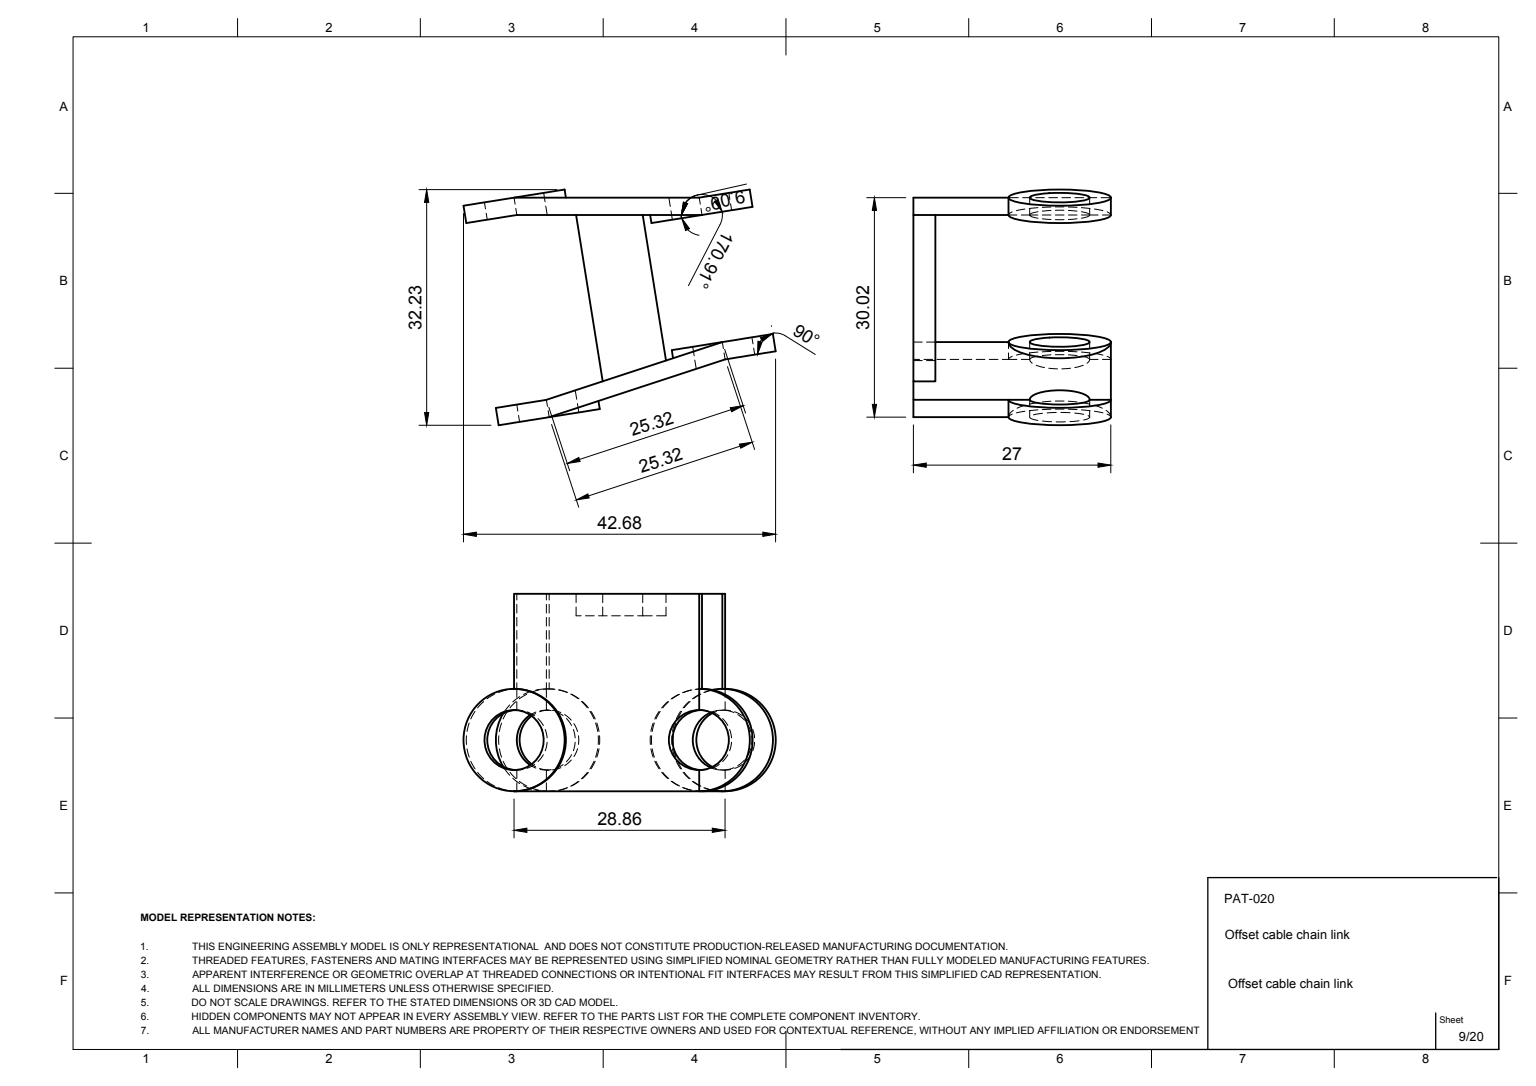
ISO-10303-21;
HEADER;
/* Generated by software containing ST-Developer
 * from STEP Tools, Inc. (www.steptools.com) 
 */

FILE_DESCRIPTION(
/* description */ ('Cable chain and bracket set'),
/* implementation_level */ '2;1');

FILE_NAME(
/* name */ 'Offset cable chain link.step',
/* time_stamp */ '2026-10-29T17:19:47-07:00',
/* author */ (''),
/* organization */ (''),
/* preprocessor_version */ 'ST-DEVELOPER v20.2',
/* originating_system */ 'Autodesk Translation Framework v15.17.0.0',
/* authorisation */ '');

FILE_SCHEMA (('AUTOMOTIVE_DESIGN { 1 0 10303 214 3 1 1 }'));
ENDSEC;

DATA;
#10=MECHANICAL_DESIGN_GEOMETRIC_PRESENTATION_REPRESENTATION('',(#338),#5929);
#291=ELLIPSE('',#3464,0.415214835958494,0.410000000000047);
#292=ELLIPSE('',#3467,0.415214835958494,0.410000000000047);
#293=ELLIPSE('',#3473,0.415214835958495,0.410000000000047);
#294=ELLIPSE('',#3475,0.415214835958495,0.410000000000047);
#295=ELLIPSE('',#3478,0.415214835958495,0.410000000000047);
#296=ELLIPSE('',#3480,0.415214835958495,0.410000000000047);
#297=ELLIPSE('',#3486,0.708903378465722,0.70000000000008);
#298=ELLIPSE('',#3488,0.708903378465722,0.70000000000008);
#299=ELLIPSE('',#3499,0.708903378465722,0.70000000000008);
#300=ELLIPSE('',#3510,0.708903378465722,0.70000000000008);
#312=SHAPE_REPRESENTATION_RELATIONSHIP('SRR','None',#6043,#325);
#325=ADVANCED_BREP_SHAPE_REPRESENTATION('',(#351),#5910);
#338=STYLED_ITEM('',(#6234),#351);
#351=MANIFOLD_SOLID_BREP('Body1',#3332);
#371=FACE_BOUND('',#751,.T.);
#372=FACE_BOUND('',#762,.T.);
#373=FACE_BOUND('',#765,.T.);
#374=FACE_BOUND('',#774,.T.);
#421=PLANE('',#3481);
#422=PLANE('',#3483);
#423=PLANE('',#3485);
#424=PLANE('',#3487);
#425=PLANE('',#3489);
#426=PLANE('',#3490);
#427=PLANE('',#3491);
#428=PLANE('',#3492);
#429=PLANE('',#3497);
#430=PLANE('',#3500);
#431=PLANE('',#3501);
#432=PLANE('',#3502);
#433=PLANE('',#3503);
#434=PLANE('',#3508);
#435=PLANE('',#3509);
#436=PLANE('',#3511);
#437=PLANE('',#3517);
#438=PLANE('',#3518);
#439=PLANE('',#3519);
#440=PLANE('',#3520);
#441=PLANE('',#3521);
#442=PLANE('',#3522);
#549=FACE_OUTER_BOUND('',#739,.T.);
#550=FACE_OUTER_BOUND('',#740,.T.);
#551=FACE_OUTER_BOUND('',#741,.T.);
#552=FACE_OUTER_BOUND('',#742,.T.);
#553=FACE_OUTER_BOUND('',#743,.T.);
#554=FACE_OUTER_BOUND('',#744,.T.);
#555=FACE_OUTER_BOUND('',#745,.T.);
#556=FACE_OUTER_BOUND('',#746,.T.);
#557=FACE_OUTER_BOUND('',#747,.T.);
#558=FACE_OUTER_BOUND('',#748,.T.);
#559=FACE_OUTER_BOUND('',#749,.T.);
#560=FACE_OUTER_BOUND('',#750,.T.);
#561=FACE_OUTER_BOUND('',#752,.T.);
#562=FACE_OUTER_BOUND('',#753,.T.);
#563=FACE_OUTER_BOUND('',#754,.T.);
#564=FACE_OUTER_BOUND('',#755,.T.);
#565=FACE_OUTER_BOUND('',#756,.T.);
#566=FACE_OUTER_BOUND('',#757,.T.);
#567=FACE_OUTER_BOUND('',#758,.T.);
#568=FACE_OUTER_BOUND('',#759,.T.);
#569=FACE_OUTER_BOUND('',#760,.T.);
#570=FACE_OUTER_BOUND('',#761,.T.);
#571=FACE_OUTER_BOUND('',#763,.T.);
#572=FACE_OUTER_BOUND('',#764,.T.);
#573=FACE_OUTER_BOUND('',#766,.T.);
#574=FACE_OUTER_BOUND('',#767,.T.);
#575=FACE_OUTER_BOUND('',#768,.T.);
#576=FACE_OUTER_BOUND('',#769,.T.);
#577=FACE_OUTER_BOUND('',#770,.T.);
#578=FACE_OUTER_BOUND('',#771,.T.);
#579=FACE_OUTER_BOUND('',#772,.T.);
#580=FACE_OUTER_BOUND('',#773,.T.);
#581=FACE_OUTER_BOUND('',#775,.T.);
#582=FACE_OUTER_BOUND('',#776,.T.);
#739=EDGE_LOOP('',(#2369,#2370,#2371,#2372,#2373,#2374));
#740=EDGE_LOOP('',(#2375,#2376,#2377,#2378,#2379,#2380));
#741=EDGE_LOOP('',(#2381,#2382,#2383,#2384,#2385,#2386));
#742=EDGE_LOOP('',(#2387,#2388,#2389,#2390,#2391,#2392));
#743=EDGE_LOOP('',(#2393,#2394,#2395,#2396,#2397));
#744=EDGE_LOOP('',(#2398,#2399,#2400,#2401,#2402));
#745=EDGE_LOOP('',(#2403,#2404,#2405,#2406,#2407,#2408,#2409,#2410,#2411));
#746=EDGE_LOOP('',(#2412,#2413,#2414,#2415,#2416,#2417,#2418,#2419,#2420));
#747=EDGE_LOOP('',(#2421,#2422,#2423,#2424));
#748=EDGE_LOOP('',(#2425,#2426,#2427,#2428));
#749=EDGE_LOOP('',(#2429,#2430,#2431,#2432));
#750=EDGE_LOOP('',(#2433,#2434));
#751=EDGE_LOOP('',(#2435));
#752=EDGE_LOOP('',(#2436,#2437,#2438,#2439));
#753=EDGE_LOOP('',(#2440,#2441,#2442,#2443));
#754=EDGE_LOOP('',(#2444,#2445));
#755=EDGE_LOOP('',(#2446,#2447,#2448,#2449,#2450,#2451,#2452,#2453,#2454,
#2455,#2456,#2457));
#756=EDGE_LOOP('',(#2458,#2459,#2460,#2461));
#757=EDGE_LOOP('',(#2462,#2463,#2464,#2465));
#758=EDGE_LOOP('',(#2466,#2467,#2468,#2469));
#759=EDGE_LOOP('',(#2470,#2471));
#760=EDGE_LOOP('',(#2472,#2473,#2474,#2475));
#761=EDGE_LOOP('',(#2476,#2477));
#762=EDGE_LOOP('',(#2478));
#763=EDGE_LOOP('',(#2479,#2480,#2481,#2482,#2483,#2484,#2485,#2486,#2487,
#2488,#2489,#2490));
#764=EDGE_LOOP('',(#2491,#2492));
#765=EDGE_LOOP('',(#2493));
#766=EDGE_LOOP('',(#2494,#2495));
#767=EDGE_LOOP('',(#2496,#2497,#2498,#2499));
#768=EDGE_LOOP('',(#2500,#2501,#2502,#2503));
#769=EDGE_LOOP('',(#2504,#2505,#2506,#2507));
#770=EDGE_LOOP('',(#2508,#2509,#2510,#2511));
#771=EDGE_LOOP('',(#2512,#2513,#2514,#2515));
#772=EDGE_LOOP('',(#2516,#2517,#2518,#2519,#2520,#2521,#2522,#2523,#2524,
#2525,#2526,#2527));
#773=EDGE_LOOP('',(#2528,#2529));
#774=EDGE_LOOP('',(#2530));
#775=EDGE_LOOP('',(#2531,#2532));
#776=EDGE_LOOP('',(#2533,#2534,#2535,#2536));
#981=LINE('',#4989,#1241);
#982=LINE('',#5002,#1242);
#983=LINE('',#5012,#1243);
#984=LINE('',#5019,#1244);
#985=LINE('',#5027,#1245);
#986=LINE('',#5030,#1246);
#987=LINE('',#5033,#1247);
#988=LINE('',#5036,#1248);
#989=LINE('',#5039,#1249);
#990=LINE('',#5041,#1250);
#991=LINE('',#5043,#1251);
#992=LINE('',#5045,#1252);
#993=LINE('',#5049,#1253);
#994=LINE('',#5050,#1254);
#995=LINE('',#5053,#1255);
#996=LINE('',#5055,#1256);
#997=LINE('',#5059,#1257);
#998=LINE('',#5061,#1258);
#999=LINE('',#5063,#1259);
#1000=LINE('',#5064,#1260);
#1001=LINE('',#5068,#1261);
#1002=LINE('',#5070,#1262);
#1003=LINE('',#5072,#1263);
#1004=LINE('',#5073,#1264);
#1005=LINE('',#5077,#1265);
#1006=LINE('',#5079,#1266);
#1007=LINE('',#5081,#1267);
#1008=LINE('',#5082,#1268);
#1009=LINE('',#5084,#1269);
#1010=LINE('',#5085,#1270);
#1011=LINE('',#5092,#1271);
#1012=LINE('',#5094,#1272);
#1013=LINE('',#5100,#1273);
#1014=LINE('',#5101,#1274);
#1015=LINE('',#5103,#1275);
#1016=LINE('',#5104,#1276);
#1017=LINE('',#5105,#1277);
#1018=LINE('',#5107,#1278);
#1019=LINE('',#5109,#1279);
#1020=LINE('',#5110,#1280);
#1021=LINE('',#5112,#1281);
#1022=LINE('',#5120,#1282);
#1023=LINE('',#5124,#1283);
#1024=LINE('',#5125,#1284);
#1025=LINE('',#5127,#1285);
#1026=LINE('',#5128,#1286);
#1027=LINE('',#5134,#1287);
#1028=LINE('',#5135,#1288);
#1029=LINE('',#5139,#1289);
#1030=LINE('',#5141,#1290);
#1031=LINE('',#5142,#1291);
#1032=LINE('',#5144,#1292);
#1241=VECTOR('',#3944,0.410000000000047);
#1242=VECTOR('',#3957,0.410000000000047);
#1243=VECTOR('',#3968,0.410000000000047);
#1244=VECTOR('',#3977,0.410000000000047);
#1245=VECTOR('',#3986,1.00000000000011);
#1246=VECTOR('',#3989,1.00000000000011);
#1247=VECTOR('',#3992,1.00000000000011);
#1248=VECTOR('',#3995,1.00000000000011);
#1249=VECTOR('',#3998,1.00000000000011);
#1250=VECTOR('',#3999,1.00000000000011);
#1251=VECTOR('',#4000,1.00000000000011);
#1252=VECTOR('',#4001,1.00000000000011);
#1253=VECTOR('',#4004,1.00000000000011);
#1254=VECTOR('',#4005,1.00000000000011);
#1255=VECTOR('',#4008,1.00000000000011);
#1256=VECTOR('',#4009,1.00000000000011);
#1257=VECTOR('',#4012,1.00000000000011);
#1258=VECTOR('',#4013,1.00000000000011);
#1259=VECTOR('',#4014,1.00000000000011);
#1260=VECTOR('',#4015,1.00000000000011);
#1261=VECTOR('',#4018,1.00000000000011);
#1262=VECTOR('',#4019,1.00000000000011);
#1263=VECTOR('',#4020,1.00000000000011);
#1264=VECTOR('',#4021,1.00000000000011);
#1265=VECTOR('',#4024,1.00000000000011);
#1266=VECTOR('',#4025,1.00000000000011);
#1267=VECTOR('',#4026,1.00000000000011);
#1268=VECTOR('',#4027,1.00000000000011);
#1269=VECTOR('',#4030,1.00000000000011);
#1270=VECTOR('',#4031,1.00000000000011);
#1271=VECTOR('',#4040,1.00000000000011);
#1272=VECTOR('',#4043,1.00000000000011);
#1273=VECTOR('',#4052,1.00000000000011);
#1274=VECTOR('',#4053,1.00000000000011);
#1275=VECTOR('',#4054,1.00000000000011);
#1276=VECTOR('',#4055,1.00000000000011);
#1277=VECTOR('',#4056,1.00000000000011);
#1278=VECTOR('',#4059,1.00000000000011);
#1279=VECTOR('',#4062,1.00000000000011);
#1280=VECTOR('',#4063,1.00000000000011);
#1281=VECTOR('',#4066,1.00000000000011);
#1282=VECTOR('',#4079,1.00000000000011);
#1283=VECTOR('',#4082,1.00000000000011);
#1284=VECTOR('',#4083,1.00000000000011);
#1285=VECTOR('',#4084,1.00000000000011);
#1286=VECTOR('',#4085,1.00000000000011);
#1287=VECTOR('',#4096,1.00000000000011);
#1288=VECTOR('',#4097,1.00000000000011);
#1289=VECTOR('',#4104,1.00000000000011);
#1290=VECTOR('',#4107,1.00000000000011);
#1291=VECTOR('',#4108,1.00000000000011);
#1292=VECTOR('',#4111,1.00000000000011);
#1465=CIRCLE('',#3462,0.410000000000047);
#1466=CIRCLE('',#3463,0.410000000000047);
#1467=CIRCLE('',#3465,0.410000000000047);
#1468=CIRCLE('',#3468,0.410000000000047);
#1469=CIRCLE('',#3469,0.410000000000047);
#1470=CIRCLE('',#3470,0.410000000000047);
#1471=CIRCLE('',#3472,0.410000000000047);
#1472=CIRCLE('',#3474,0.410000000000047);
#1473=CIRCLE('',#3477,0.410000000000047);
#1474=CIRCLE('',#3479,0.410000000000047);
#1475=CIRCLE('',#3482,0.70000000000008);
#1476=CIRCLE('',#3484,0.70000000000008);
#1477=CIRCLE('',#3493,0.70000000000008);
#1478=CIRCLE('',#3494,0.70000000000008);
#1479=CIRCLE('',#3496,0.70000000000008);
#1480=CIRCLE('',#3505,0.70000000000008);
#1481=CIRCLE('',#3507,0.70000000000008);
#1482=CIRCLE('',#3512,0.70000000000008);
#1483=CIRCLE('',#3513,0.70000000000008);
#1484=CIRCLE('',#3516,0.70000000000008);
#1485=CIRCLE('',#3523,0.70000000000008);
#1486=CIRCLE('',#3524,0.70000000000008);
#1601=VERTEX_POINT('',#4986);
#1602=VERTEX_POINT('',#4988);
#1603=VERTEX_POINT('',#4990);
#1604=VERTEX_POINT('',#4992);
#1605=VERTEX_POINT('',#4996);
#1606=VERTEX_POINT('',#4997);
#1607=VERTEX_POINT('',#4999);
#1608=VERTEX_POINT('',#5001);
#1609=VERTEX_POINT('',#5006);
#1610=VERTEX_POINT('',#5007);
#1611=VERTEX_POINT('',#5009);
#1612=VERTEX_POINT('',#5011);
#1613=VERTEX_POINT('',#5016);
#1614=VERTEX_POINT('',#5018);
#1615=VERTEX_POINT('',#5020);
#1616=VERTEX_POINT('',#5022);
#1617=VERTEX_POINT('',#5026);
#1618=VERTEX_POINT('',#5028);
#1619=VERTEX_POINT('',#5032);
#1620=VERTEX_POINT('',#5034);
#1621=VERTEX_POINT('',#5038);
#1622=VERTEX_POINT('',#5040);
#1623=VERTEX_POINT('',#5042);
#1624=VERTEX_POINT('',#5044);
#1625=VERTEX_POINT('',#5046);
#1626=VERTEX_POINT('',#5048);
#1627=VERTEX_POINT('',#5052);
#1628=VERTEX_POINT('',#5054);
#1629=VERTEX_POINT('',#5056);
#1630=VERTEX_POINT('',#5058);
#1631=VERTEX_POINT('',#5060);
#1632=VERTEX_POINT('',#5062);
#1633=VERTEX_POINT('',#5066);
#1634=VERTEX_POINT('',#5067);
#1635=VERTEX_POINT('',#5069);
#1636=VERTEX_POINT('',#5071);
#1637=VERTEX_POINT('',#5075);
#1638=VERTEX_POINT('',#5076);
#1639=VERTEX_POINT('',#5078);
#1640=VERTEX_POINT('',#5080);
#1641=VERTEX_POINT('',#5087);
#1642=VERTEX_POINT('',#5088);
#1643=VERTEX_POINT('',#5099);
#1644=VERTEX_POINT('',#5102);
#1645=VERTEX_POINT('',#5119);
#1646=VERTEX_POINT('',#5121);
#1647=VERTEX_POINT('',#5123);
#1648=VERTEX_POINT('',#5126);
#1885=EDGE_CURVE('',#1601,#1601,#1465,.T.);
#1886=EDGE_CURVE('',#1601,#1602,#981,.T.);
#1887=EDGE_CURVE('',#1603,#1602,#1466,.T.);
#1888=EDGE_CURVE('',#1604,#1603,#291,.T.);
#1889=EDGE_CURVE('',#1602,#1604,#1467,.T.);
#1890=EDGE_CURVE('',#1605,#1606,#292,.T.);
#1891=EDGE_CURVE('',#1607,#1605,#1468,.T.);
#1892=EDGE_CURVE('',#1607,#1608,#982,.T.);
#1893=EDGE_CURVE('',#1608,#1608,#1469,.T.);
#1894=EDGE_CURVE('',#1606,#1607,#1470,.T.);
#1895=EDGE_CURVE('',#1609,#1610,#1471,.T.);
#1896=EDGE_CURVE('',#1611,#1609,#293,.T.);
#1897=EDGE_CURVE('',#1611,#1612,#983,.T.);
#1898=EDGE_CURVE('',#1612,#1612,#1472,.T.);
#1899=EDGE_CURVE('',#1610,#1611,#294,.T.);
#1900=EDGE_CURVE('',#1613,#1613,#1473,.T.);
#1901=EDGE_CURVE('',#1613,#1614,#984,.T.);
#1902=EDGE_CURVE('',#1615,#1614,#295,.T.);
#1903=EDGE_CURVE('',#1616,#1615,#1474,.T.);
#1904=EDGE_CURVE('',#1614,#1616,#296,.T.);
#1905=EDGE_CURVE('',#1605,#1617,#985,.T.);
#1906=EDGE_CURVE('',#1618,#1617,#1475,.T.);
#1907=EDGE_CURVE('',#1618,#1606,#986,.T.);
#1908=EDGE_CURVE('',#1604,#1619,#987,.T.);
#1909=EDGE_CURVE('',#1619,#1620,#1476,.T.);
#1910=EDGE_CURVE('',#1620,#1603,#988,.T.);
#1911=EDGE_CURVE('',#1621,#1616,#989,.T.);
#1912=EDGE_CURVE('',#1622,#1621,#990,.T.);
#1913=EDGE_CURVE('',#1622,#1623,#991,.T.);
#1914=EDGE_CURVE('',#1623,#1624,#992,.T.);
#1915=EDGE_CURVE('',#1625,#1624,#297,.T.);
#1916=EDGE_CURVE('',#1626,#1625,#993,.T.);
#1917=EDGE_CURVE('',#1615,#1626,#994,.T.);
#1918=EDGE_CURVE('',#1609,#1627,#995,.T.);
#1919=EDGE_CURVE('',#1628,#1627,#996,.T.);
#1920=EDGE_CURVE('',#1629,#1628,#298,.T.);
#1921=EDGE_CURVE('',#1630,#1629,#997,.T.);
#1922=EDGE_CURVE('',#1630,#1631,#998,.T.);
#1923=EDGE_CURVE('',#1631,#1632,#999,.T.);
#1924=EDGE_CURVE('',#1632,#1610,#1000,.T.);
#1925=EDGE_CURVE('',#1633,#1634,#1001,.T.);
#1926=EDGE_CURVE('',#1635,#1633,#1002,.T.);
#1927=EDGE_CURVE('',#1636,#1635,#1003,.T.);
#1928=EDGE_CURVE('',#1636,#1634,#1004,.T.);
#1929=EDGE_CURVE('',#1637,#1638,#1005,.T.);
#1930=EDGE_CURVE('',#1637,#1639,#1006,.T.);
#1931=EDGE_CURVE('',#1640,#1639,#1007,.T.);
#1932=EDGE_CURVE('',#1638,#1640,#1008,.T.);
#1933=EDGE_CURVE('',#1638,#1633,#1009,.T.);
#1934=EDGE_CURVE('',#1635,#1640,#1010,.T.);
#1935=EDGE_CURVE('',#1641,#1642,#1477,.T.);
#1936=EDGE_CURVE('',#1642,#1641,#1478,.T.);
#1937=EDGE_CURVE('',#1621,#1641,#1011,.T.);
#1938=EDGE_CURVE('',#1626,#1621,#1479,.T.);
#1939=EDGE_CURVE('',#1642,#1626,#1012,.T.);
#1940=EDGE_CURVE('',#1641,#1642,#299,.T.);
#1941=EDGE_CURVE('',#1643,#1618,#1013,.T.);
#1942=EDGE_CURVE('',#1643,#1636,#1014,.T.);
#1943=EDGE_CURVE('',#1639,#1644,#1015,.T.);
#1944=EDGE_CURVE('',#1644,#1641,#1016,.T.);
#1945=EDGE_CURVE('',#1617,#1642,#1017,.T.);
#1946=EDGE_CURVE('',#1644,#1622,#1018,.T.);
#1947=EDGE_CURVE('',#1624,#1618,#1019,.T.);
#1948=EDGE_CURVE('',#1623,#1643,#1020,.T.);
#1949=EDGE_CURVE('',#1617,#1625,#1021,.T.);
#1950=EDGE_CURVE('',#1625,#1624,#1480,.T.);
#1951=EDGE_CURVE('',#1624,#1625,#1481,.T.);
#1952=EDGE_CURVE('',#1645,#1620,#1022,.T.);
#1953=EDGE_CURVE('',#1645,#1646,#300,.T.);
#1954=EDGE_CURVE('',#1647,#1646,#1023,.T.);
#1955=EDGE_CURVE('',#1647,#1637,#1024,.T.);
#1956=EDGE_CURVE('',#1634,#1648,#1025,.T.);
#1957=EDGE_CURVE('',#1648,#1619,#1026,.T.);
#1958=EDGE_CURVE('',#1645,#1646,#1482,.T.);
#1959=EDGE_CURVE('',#1646,#1645,#1483,.T.);
#1960=EDGE_CURVE('',#1646,#1632,#1027,.T.);
#1961=EDGE_CURVE('',#1627,#1645,#1028,.T.);
#1962=EDGE_CURVE('',#1627,#1632,#1484,.T.);
#1963=EDGE_CURVE('',#1631,#1647,#1029,.T.);
#1964=EDGE_CURVE('',#1619,#1629,#1030,.T.);
#1965=EDGE_CURVE('',#1648,#1630,#1031,.T.);
#1966=EDGE_CURVE('',#1628,#1620,#1032,.T.);
#1967=EDGE_CURVE('',#1628,#1629,#1485,.T.);
#1968=EDGE_CURVE('',#1629,#1628,#1486,.T.);
#2369=ORIENTED_EDGE('',*,*,#1885,.F.);
#2370=ORIENTED_EDGE('',*,*,#1886,.T.);
#2371=ORIENTED_EDGE('',*,*,#1887,.F.);
#2372=ORIENTED_EDGE('',*,*,#1888,.F.);
#2373=ORIENTED_EDGE('',*,*,#1889,.F.);
#2374=ORIENTED_EDGE('',*,*,#1886,.F.);
#2375=ORIENTED_EDGE('',*,*,#1890,.F.);
#2376=ORIENTED_EDGE('',*,*,#1891,.F.);
#2377=ORIENTED_EDGE('',*,*,#1892,.T.);
#2378=ORIENTED_EDGE('',*,*,#1893,.F.);
#2379=ORIENTED_EDGE('',*,*,#1892,.F.);
#2380=ORIENTED_EDGE('',*,*,#1894,.F.);
#2381=ORIENTED_EDGE('',*,*,#1895,.F.);
#2382=ORIENTED_EDGE('',*,*,#1896,.F.);
#2383=ORIENTED_EDGE('',*,*,#1897,.T.);
#2384=ORIENTED_EDGE('',*,*,#1898,.F.);
#2385=ORIENTED_EDGE('',*,*,#1897,.F.);
#2386=ORIENTED_EDGE('',*,*,#1899,.F.);
#2387=ORIENTED_EDGE('',*,*,#1900,.F.);
#2388=ORIENTED_EDGE('',*,*,#1901,.T.);
#2389=ORIENTED_EDGE('',*,*,#1902,.F.);
#2390=ORIENTED_EDGE('',*,*,#1903,.F.);
#2391=ORIENTED_EDGE('',*,*,#1904,.F.);
#2392=ORIENTED_EDGE('',*,*,#1901,.F.);
#2393=ORIENTED_EDGE('',*,*,#1894,.T.);
#2394=ORIENTED_EDGE('',*,*,#1891,.T.);
#2395=ORIENTED_EDGE('',*,*,#1905,.T.);
#2396=ORIENTED_EDGE('',*,*,#1906,.F.);
#2397=ORIENTED_EDGE('',*,*,#1907,.T.);
#2398=ORIENTED_EDGE('',*,*,#1887,.T.);
#2399=ORIENTED_EDGE('',*,*,#1889,.T.);
#2400=ORIENTED_EDGE('',*,*,#1908,.T.);
#2401=ORIENTED_EDGE('',*,*,#1909,.T.);
#2402=ORIENTED_EDGE('',*,*,#1910,.T.);
#2403=ORIENTED_EDGE('',*,*,#1902,.T.);
#2404=ORIENTED_EDGE('',*,*,#1904,.T.);
#2405=ORIENTED_EDGE('',*,*,#1911,.F.);
#2406=ORIENTED_EDGE('',*,*,#1912,.F.);
#2407=ORIENTED_EDGE('',*,*,#1913,.T.);
#2408=ORIENTED_EDGE('',*,*,#1914,.T.);
#2409=ORIENTED_EDGE('',*,*,#1915,.F.);
#2410=ORIENTED_EDGE('',*,*,#1916,.F.);
#2411=ORIENTED_EDGE('',*,*,#1917,.F.);
#2412=ORIENTED_EDGE('',*,*,#1899,.T.);
#2413=ORIENTED_EDGE('',*,*,#1896,.T.);
#2414=ORIENTED_EDGE('',*,*,#1918,.T.);
#2415=ORIENTED_EDGE('',*,*,#1919,.F.);
#2416=ORIENTED_EDGE('',*,*,#1920,.F.);
#2417=ORIENTED_EDGE('',*,*,#1921,.F.);
#2418=ORIENTED_EDGE('',*,*,#1922,.T.);
#2419=ORIENTED_EDGE('',*,*,#1923,.T.);
#2420=ORIENTED_EDGE('',*,*,#1924,.T.);
#2421=ORIENTED_EDGE('',*,*,#1925,.F.);
#2422=ORIENTED_EDGE('',*,*,#1926,.F.);
#2423=ORIENTED_EDGE('',*,*,#1927,.F.);
#2424=ORIENTED_EDGE('',*,*,#1928,.T.);
#2425=ORIENTED_EDGE('',*,*,#1929,.F.);
#2426=ORIENTED_EDGE('',*,*,#1930,.T.);
#2427=ORIENTED_EDGE('',*,*,#1931,.F.);
#2428=ORIENTED_EDGE('',*,*,#1932,.F.);
#2429=ORIENTED_EDGE('',*,*,#1933,.F.);
#2430=ORIENTED_EDGE('',*,*,#1932,.T.);
#2431=ORIENTED_EDGE('',*,*,#1934,.F.);
#2432=ORIENTED_EDGE('',*,*,#1926,.T.);
#2433=ORIENTED_EDGE('',*,*,#1935,.F.);
#2434=ORIENTED_EDGE('',*,*,#1936,.F.);
#2435=ORIENTED_EDGE('',*,*,#1900,.T.);
#2436=ORIENTED_EDGE('',*,*,#1937,.F.);
#2437=ORIENTED_EDGE('',*,*,#1938,.F.);
#2438=ORIENTED_EDGE('',*,*,#1939,.F.);
#2439=ORIENTED_EDGE('',*,*,#1936,.T.);
#2440=ORIENTED_EDGE('',*,*,#1903,.T.);
#2441=ORIENTED_EDGE('',*,*,#1917,.T.);
#2442=ORIENTED_EDGE('',*,*,#1938,.T.);
#2443=ORIENTED_EDGE('',*,*,#1911,.T.);
#2444=ORIENTED_EDGE('',*,*,#1940,.F.);
#2445=ORIENTED_EDGE('',*,*,#1935,.T.);
#2446=ORIENTED_EDGE('',*,*,#1890,.T.);
#2447=ORIENTED_EDGE('',*,*,#1907,.F.);
#2448=ORIENTED_EDGE('',*,*,#1941,.F.);
#2449=ORIENTED_EDGE('',*,*,#1942,.T.);
#2450=ORIENTED_EDGE('',*,*,#1927,.T.);
#2451=ORIENTED_EDGE('',*,*,#1934,.T.);
#2452=ORIENTED_EDGE('',*,*,#1931,.T.);
#2453=ORIENTED_EDGE('',*,*,#1943,.T.);
#2454=ORIENTED_EDGE('',*,*,#1944,.T.);
#2455=ORIENTED_EDGE('',*,*,#1940,.T.);
#2456=ORIENTED_EDGE('',*,*,#1945,.F.);
#2457=ORIENTED_EDGE('',*,*,#1905,.F.);
#2458=ORIENTED_EDGE('',*,*,#1937,.T.);
#2459=ORIENTED_EDGE('',*,*,#1944,.F.);
#2460=ORIENTED_EDGE('',*,*,#1946,.T.);
#2461=ORIENTED_EDGE('',*,*,#1912,.T.);
#2462=ORIENTED_EDGE('',*,*,#1947,.F.);
#2463=ORIENTED_EDGE('',*,*,#1914,.F.);
#2464=ORIENTED_EDGE('',*,*,#1948,.T.);
#2465=ORIENTED_EDGE('',*,*,#1941,.T.);
#2466=ORIENTED_EDGE('',*,*,#1949,.F.);
#2467=ORIENTED_EDGE('',*,*,#1945,.T.);
#2468=ORIENTED_EDGE('',*,*,#1939,.T.);
#2469=ORIENTED_EDGE('',*,*,#1916,.T.);
#2470=ORIENTED_EDGE('',*,*,#1915,.T.);
#2471=ORIENTED_EDGE('',*,*,#1950,.F.);
#2472=ORIENTED_EDGE('',*,*,#1949,.T.);
#2473=ORIENTED_EDGE('',*,*,#1951,.F.);
#2474=ORIENTED_EDGE('',*,*,#1947,.T.);
#2475=ORIENTED_EDGE('',*,*,#1906,.T.);
#2476=ORIENTED_EDGE('',*,*,#1950,.T.);
#2477=ORIENTED_EDGE('',*,*,#1951,.T.);
#2478=ORIENTED_EDGE('',*,*,#1893,.T.);
#2479=ORIENTED_EDGE('',*,*,#1888,.T.);
#2480=ORIENTED_EDGE('',*,*,#1910,.F.);
#2481=ORIENTED_EDGE('',*,*,#1952,.F.);
#2482=ORIENTED_EDGE('',*,*,#1953,.T.);
#2483=ORIENTED_EDGE('',*,*,#1954,.F.);
#2484=ORIENTED_EDGE('',*,*,#1955,.T.);
#2485=ORIENTED_EDGE('',*,*,#1929,.T.);
#2486=ORIENTED_EDGE('',*,*,#1933,.T.);
#2487=ORIENTED_EDGE('',*,*,#1925,.T.);
#2488=ORIENTED_EDGE('',*,*,#1956,.T.);
#2489=ORIENTED_EDGE('',*,*,#1957,.T.);
#2490=ORIENTED_EDGE('',*,*,#1908,.F.);
#2491=ORIENTED_EDGE('',*,*,#1958,.T.);
#2492=ORIENTED_EDGE('',*,*,#1959,.T.);
#2493=ORIENTED_EDGE('',*,*,#1898,.T.);
#2494=ORIENTED_EDGE('',*,*,#1953,.F.);
#2495=ORIENTED_EDGE('',*,*,#1959,.F.);
#2496=ORIENTED_EDGE('',*,*,#1960,.F.);
#2497=ORIENTED_EDGE('',*,*,#1958,.F.);
#2498=ORIENTED_EDGE('',*,*,#1961,.F.);
#2499=ORIENTED_EDGE('',*,*,#1962,.T.);
#2500=ORIENTED_EDGE('',*,*,#1895,.T.);
#2501=ORIENTED_EDGE('',*,*,#1924,.F.);
#2502=ORIENTED_EDGE('',*,*,#1962,.F.);
#2503=ORIENTED_EDGE('',*,*,#1918,.F.);
#2504=ORIENTED_EDGE('',*,*,#1960,.T.);
#2505=ORIENTED_EDGE('',*,*,#1923,.F.);
#2506=ORIENTED_EDGE('',*,*,#1963,.T.);
#2507=ORIENTED_EDGE('',*,*,#1954,.T.);
#2508=ORIENTED_EDGE('',*,*,#1964,.F.);
#2509=ORIENTED_EDGE('',*,*,#1957,.F.);
#2510=ORIENTED_EDGE('',*,*,#1965,.T.);
#2511=ORIENTED_EDGE('',*,*,#1921,.T.);
#2512=ORIENTED_EDGE('',*,*,#1966,.F.);
#2513=ORIENTED_EDGE('',*,*,#1919,.T.);
#2514=ORIENTED_EDGE('',*,*,#1961,.T.);
#2515=ORIENTED_EDGE('',*,*,#1952,.T.);
#2516=ORIENTED_EDGE('',*,*,#1955,.F.);
#2517=ORIENTED_EDGE('',*,*,#1963,.F.);
#2518=ORIENTED_EDGE('',*,*,#1922,.F.);
#2519=ORIENTED_EDGE('',*,*,#1965,.F.);
#2520=ORIENTED_EDGE('',*,*,#1956,.F.);
#2521=ORIENTED_EDGE('',*,*,#1928,.F.);
#2522=ORIENTED_EDGE('',*,*,#1942,.F.);
#2523=ORIENTED_EDGE('',*,*,#1948,.F.);
#2524=ORIENTED_EDGE('',*,*,#1913,.F.);
#2525=ORIENTED_EDGE('',*,*,#1946,.F.);
#2526=ORIENTED_EDGE('',*,*,#1943,.F.);
#2527=ORIENTED_EDGE('',*,*,#1930,.F.);
#2528=ORIENTED_EDGE('',*,*,#1967,.F.);
#2529=ORIENTED_EDGE('',*,*,#1968,.F.);
#2530=ORIENTED_EDGE('',*,*,#1885,.T.);
#2531=ORIENTED_EDGE('',*,*,#1920,.T.);
#2532=ORIENTED_EDGE('',*,*,#1967,.T.);
#2533=ORIENTED_EDGE('',*,*,#1964,.T.);
#2534=ORIENTED_EDGE('',*,*,#1968,.T.);
#2535=ORIENTED_EDGE('',*,*,#1966,.T.);
#2536=ORIENTED_EDGE('',*,*,#1909,.F.);
#3103=CYLINDRICAL_SURFACE('',#3461,0.410000000000047);
#3104=CYLINDRICAL_SURFACE('',#3466,0.410000000000047);
#3105=CYLINDRICAL_SURFACE('',#3471,0.410000000000047);
#3106=CYLINDRICAL_SURFACE('',#3476,0.410000000000047);
#3107=CYLINDRICAL_SURFACE('',#3495,0.70000000000008);
#3108=CYLINDRICAL_SURFACE('',#3498,0.70000000000008);
#3109=CYLINDRICAL_SURFACE('',#3504,0.70000000000008);
#3110=CYLINDRICAL_SURFACE('',#3506,0.70000000000008);
#3111=CYLINDRICAL_SURFACE('',#3514,0.70000000000008);
#3112=CYLINDRICAL_SURFACE('',#3515,0.70000000000008);
#3113=CYLINDRICAL_SURFACE('',#3525,0.70000000000008);
#3114=CYLINDRICAL_SURFACE('',#3526,0.70000000000008);
#3171=ADVANCED_FACE('',(#549),#3103,.F.);
#3172=ADVANCED_FACE('',(#550),#3104,.F.);
#3173=ADVANCED_FACE('',(#551),#3105,.F.);
#3174=ADVANCED_FACE('',(#552),#3106,.F.);
#3175=ADVANCED_FACE('',(#553),#421,.F.);
#3176=ADVANCED_FACE('',(#554),#422,.T.);
#3177=ADVANCED_FACE('',(#555),#423,.T.);
#3178=ADVANCED_FACE('',(#556),#424,.T.);
#3179=ADVANCED_FACE('',(#557),#425,.T.);
#3180=ADVANCED_FACE('',(#558),#426,.T.);
#3181=ADVANCED_FACE('',(#559),#427,.T.);
#3182=ADVANCED_FACE('',(#560,#371),#428,.F.);
#3183=ADVANCED_FACE('',(#561),#3107,.T.);
#3184=ADVANCED_FACE('',(#562),#429,.T.);
#3185=ADVANCED_FACE('',(#563),#3108,.T.);
#3186=ADVANCED_FACE('',(#564),#430,.T.);
#3187=ADVANCED_FACE('',(#565),#431,.T.);
#3188=ADVANCED_FACE('',(#566),#432,.T.);
#3189=ADVANCED_FACE('',(#567),#433,.T.);
#3190=ADVANCED_FACE('',(#568),#3109,.T.);
#3191=ADVANCED_FACE('',(#569),#3110,.T.);
#3192=ADVANCED_FACE('',(#570,#372),#434,.T.);
#3193=ADVANCED_FACE('',(#571),#435,.T.);
#3194=ADVANCED_FACE('',(#572,#373),#436,.T.);
#3195=ADVANCED_FACE('',(#573),#3111,.T.);
#3196=ADVANCED_FACE('',(#574),#3112,.T.);
#3197=ADVANCED_FACE('',(#575),#437,.F.);
#3198=ADVANCED_FACE('',(#576),#438,.T.);
#3199=ADVANCED_FACE('',(#577),#439,.T.);
#3200=ADVANCED_FACE('',(#578),#440,.T.);
#3201=ADVANCED_FACE('',(#579),#441,.F.);
#3202=ADVANCED_FACE('',(#580,#374),#442,.F.);
#3203=ADVANCED_FACE('',(#581),#3113,.T.);
#3204=ADVANCED_FACE('',(#582),#3114,.T.);
#3332=CLOSED_SHELL('',(#3171,#3172,#3173,#3174,#3175,#3176,#3177,#3178,
#3179,#3180,#3181,#3182,#3183,#3184,#3185,#3186,#3187,#3188,#3189,#3190,
#3191,#3192,#3193,#3194,#3195,#3196,#3197,#3198,#3199,#3200,#3201,#3202,
#3203,#3204));
#3460=AXIS2_PLACEMENT_3D('',#4984,#3938,#3939);
#3461=AXIS2_PLACEMENT_3D('',#4985,#3940,#3941);
#3462=AXIS2_PLACEMENT_3D('',#4987,#3942,#3943);
#3463=AXIS2_PLACEMENT_3D('',#4991,#3945,#3946);
#3464=AXIS2_PLACEMENT_3D('',#4993,#3947,#3948);
#3465=AXIS2_PLACEMENT_3D('',#4994,#3949,#3950);
#3466=AXIS2_PLACEMENT_3D('',#4995,#3951,#3952);
#3467=AXIS2_PLACEMENT_3D('',#4998,#3953,#3954);
#3468=AXIS2_PLACEMENT_3D('',#5000,#3955,#3956);
#3469=AXIS2_PLACEMENT_3D('',#5003,#3958,#3959);
#3470=AXIS2_PLACEMENT_3D('',#5004,#3960,#3961);
#3471=AXIS2_PLACEMENT_3D('',#5005,#3962,#3963);
#3472=AXIS2_PLACEMENT_3D('',#5008,#3964,#3965);
#3473=AXIS2_PLACEMENT_3D('',#5010,#3966,#3967);
#3474=AXIS2_PLACEMENT_3D('',#5013,#3969,#3970);
#3475=AXIS2_PLACEMENT_3D('',#5014,#3971,#3972);
#3476=AXIS2_PLACEMENT_3D('',#5015,#3973,#3974);
#3477=AXIS2_PLACEMENT_3D('',#5017,#3975,#3976);
#3478=AXIS2_PLACEMENT_3D('',#5021,#3978,#3979);
#3479=AXIS2_PLACEMENT_3D('',#5023,#3980,#3981);
#3480=AXIS2_PLACEMENT_3D('',#5024,#3982,#3983);
#3481=AXIS2_PLACEMENT_3D('',#5025,#3984,#3985);
#3482=AXIS2_PLACEMENT_3D('',#5029,#3987,#3988);
#3483=AXIS2_PLACEMENT_3D('',#5031,#3990,#3991);
#3484=AXIS2_PLACEMENT_3D('',#5035,#3993,#3994);
#3485=AXIS2_PLACEMENT_3D('',#5037,#3996,#3997);
#3486=AXIS2_PLACEMENT_3D('',#5047,#4002,#4003);
#3487=AXIS2_PLACEMENT_3D('',#5051,#4006,#4007);
#3488=AXIS2_PLACEMENT_3D('',#5057,#4010,#4011);
#3489=AXIS2_PLACEMENT_3D('',#5065,#4016,#4017);
#3490=AXIS2_PLACEMENT_3D('',#5074,#4022,#4023);
#3491=AXIS2_PLACEMENT_3D('',#5083,#4028,#4029);
#3492=AXIS2_PLACEMENT_3D('',#5086,#4032,#4033);
#3493=AXIS2_PLACEMENT_3D('',#5089,#4034,#4035);
#3494=AXIS2_PLACEMENT_3D('',#5090,#4036,#4037);
#3495=AXIS2_PLACEMENT_3D('',#5091,#4038,#4039);
#3496=AXIS2_PLACEMENT_3D('',#5093,#4041,#4042);
#3497=AXIS2_PLACEMENT_3D('',#5095,#4044,#4045);
#3498=AXIS2_PLACEMENT_3D('',#5096,#4046,#4047);
#3499=AXIS2_PLACEMENT_3D('',#5097,#4048,#4049);
#3500=AXIS2_PLACEMENT_3D('',#5098,#4050,#4051);
#3501=AXIS2_PLACEMENT_3D('',#5106,#4057,#4058);
#3502=AXIS2_PLACEMENT_3D('',#5108,#4060,#4061);
#3503=AXIS2_PLACEMENT_3D('',#5111,#4064,#4065);
#3504=AXIS2_PLACEMENT_3D('',#5113,#4067,#4068);
#3505=AXIS2_PLACEMENT_3D('',#5114,#4069,#4070);
#3506=AXIS2_PLACEMENT_3D('',#5115,#4071,#4072);
#3507=AXIS2_PLACEMENT_3D('',#5116,#4073,#4074);
#3508=AXIS2_PLACEMENT_3D('',#5117,#4075,#4076);
#3509=AXIS2_PLACEMENT_3D('',#5118,#4077,#4078);
#3510=AXIS2_PLACEMENT_3D('',#5122,#4080,#4081);
#3511=AXIS2_PLACEMENT_3D('',#5129,#4086,#4087);
#3512=AXIS2_PLACEMENT_3D('',#5130,#4088,#4089);
#3513=AXIS2_PLACEMENT_3D('',#5131,#4090,#4091);
#3514=AXIS2_PLACEMENT_3D('',#5132,#4092,#4093);
#3515=AXIS2_PLACEMENT_3D('',#5133,#4094,#4095);
#3516=AXIS2_PLACEMENT_3D('',#5136,#4098,#4099);
#3517=AXIS2_PLACEMENT_3D('',#5137,#4100,#4101);
#3518=AXIS2_PLACEMENT_3D('',#5138,#4102,#4103);
#3519=AXIS2_PLACEMENT_3D('',#5140,#4105,#4106);
#3520=AXIS2_PLACEMENT_3D('',#5143,#4109,#4110);
#3521=AXIS2_PLACEMENT_3D('',#5145,#4112,#4113);
#3522=AXIS2_PLACEMENT_3D('',#5146,#4114,#4115);
#3523=AXIS2_PLACEMENT_3D('',#5147,#4116,#4117);
#3524=AXIS2_PLACEMENT_3D('',#5148,#4118,#4119);
#3525=AXIS2_PLACEMENT_3D('',#5149,#4120,#4121);
#3526=AXIS2_PLACEMENT_3D('',#5150,#4122,#4123);
#3938=DIRECTION('axis',(0.,0.,1.));
#3939=DIRECTION('refdir',(1.,0.,0.));
#3940=DIRECTION('center_axis',(-6.12323399573548E-17,1.,4.78224871431377E-30));
#3941=DIRECTION('ref_axis',(0.939692587475203,5.75395759716863E-17,0.342020234846066));
#3942=DIRECTION('center_axis',(-6.12323399573548E-17,1.,4.78224871431377E-30));
#3943=DIRECTION('ref_axis',(0.939692587475203,5.75395759716863E-17,0.342020234846066));
#3944=DIRECTION('',(-6.12323399573548E-17,1.,4.78224871431377E-30));
#3945=DIRECTION('center_axis',(6.12323399573548E-17,-1.,-4.78224871431377E-30));
#3946=DIRECTION('ref_axis',(0.939692587475203,5.75395759716863E-17,0.342020234846066));
#3947=DIRECTION('center_axis',(0.148462502781433,-0.987440631916705,0.0540359482919519));
#3948=DIRECTION('ref_axis',(0.927890642383958,0.157990501106673,0.337724676824699));
#3949=DIRECTION('center_axis',(6.12323399573548E-17,-1.,-4.78224871431377E-30));
#3950=DIRECTION('ref_axis',(0.939692587475203,5.75395759716863E-17,0.342020234846066));
#3951=DIRECTION('center_axis',(-6.12323399573548E-17,1.,4.78224871431377E-30));
#3952=DIRECTION('ref_axis',(0.939692587475203,5.75395759716863E-17,0.342020234846066));
#3953=DIRECTION('center_axis',(0.148462502781433,0.987440631916705,0.0540359482919519));
#3954=DIRECTION('ref_axis',(0.927890642383958,-0.157990501106673,0.337724676824699));
#3955=DIRECTION('center_axis',(-6.12323399573548E-17,1.,4.78224871431377E-30));
#3956=DIRECTION('ref_axis',(0.939692587475203,5.75395759716863E-17,0.342020234846066));
#3957=DIRECTION('',(-6.12323399573548E-17,1.,4.78224871431377E-30));
#3958=DIRECTION('center_axis',(6.12323399573548E-17,-1.,-4.78224871431377E-30));
#3959=DIRECTION('ref_axis',(0.939692587475203,5.75395759716863E-17,0.342020234846066));
#3960=DIRECTION('center_axis',(-6.12323399573548E-17,1.,4.78224871431377E-30));
#3961=DIRECTION('ref_axis',(0.939692587475203,5.75395759716863E-17,0.342020234846066));
#3962=DIRECTION('center_axis',(-6.12323399573548E-17,1.,4.78224871431377E-30));
#3963=DIRECTION('ref_axis',(0.939692587475203,5.75395759716863E-17,0.342020234846066));
#3964=DIRECTION('center_axis',(-6.12323399573548E-17,1.,4.78224871431377E-30));
#3965=DIRECTION('ref_axis',(0.939692587475203,5.75395759716863E-17,0.342020234846066));
#3966=DIRECTION('center_axis',(-0.148462502781433,0.987440631916705,-0.0540359482919519));
#3967=DIRECTION('ref_axis',(0.927890642383958,0.157990501106673,0.337724676824699));
#3968=DIRECTION('',(-6.12323399573548E-17,1.,4.78224871431377E-30));
#3969=DIRECTION('center_axis',(6.12323399573548E-17,-1.,-4.78224871431377E-30));
#3970=DIRECTION('ref_axis',(0.939692587475203,5.75395759716863E-17,0.342020234846066));
#3971=DIRECTION('center_axis',(-0.148462502781433,0.987440631916705,-0.0540359482919519));
#3972=DIRECTION('ref_axis',(0.927890642383958,0.157990501106673,0.337724676824699));
#3973=DIRECTION('center_axis',(-6.12323399573548E-17,1.,4.78224871431377E-30));
#3974=DIRECTION('ref_axis',(0.939692587475203,5.75395759716863E-17,0.342020234846066));
#3975=DIRECTION('center_axis',(-6.12323399573548E-17,1.,4.78224871431377E-30));
#3976=DIRECTION('ref_axis',(0.939692587475203,5.75395759716863E-17,0.342020234846066));
#3977=DIRECTION('',(-6.12323399573548E-17,1.,4.78224871431377E-30));
#3978=DIRECTION('center_axis',(-0.148462502781433,-0.987440631916705,-0.0540359482919519));
#3979=DIRECTION('ref_axis',(0.927890642383958,-0.157990501106673,0.337724676824699));
#3980=DIRECTION('center_axis',(6.12323399573548E-17,-1.,-4.78224871431377E-30));
#3981=DIRECTION('ref_axis',(0.939692587475203,5.75395759716863E-17,0.342020234846066));
#3982=DIRECTION('center_axis',(-0.148462502781433,-0.987440631916705,-0.0540359482919519));
#3983=DIRECTION('ref_axis',(0.927890642383958,-0.157990501106673,0.337724676824699));
#3984=DIRECTION('center_axis',(-6.12323399573548E-17,1.,4.78224871431377E-30));
#3985=DIRECTION('ref_axis',(0.939692587475203,5.75395759716863E-17,0.342020234846066));
#3986=DIRECTION('',(-0.342020234846066,-2.09426992923931E-17,0.939692587475203));
#3987=DIRECTION('center_axis',(-6.12323399573548E-17,1.,4.78224871431377E-30));
#3988=DIRECTION('ref_axis',(0.939692587475203,5.75395759716863E-17,0.342020234846066));
#3989=DIRECTION('',(-0.342020234846066,-2.09426992923931E-17,0.939692587475203));
#3990=DIRECTION('center_axis',(-6.12323399573548E-17,1.,4.78224871431377E-30));
#3991=DIRECTION('ref_axis',(0.939692587475203,5.75395759716863E-17,0.342020234846066));
#3992=DIRECTION('',(0.342020234846066,2.09426992923931E-17,-0.939692587475203));
#3993=DIRECTION('center_axis',(-6.12323399573548E-17,1.,4.78224871431377E-30));
#3994=DIRECTION('ref_axis',(0.939692587475203,5.75395759716863E-17,0.342020234846066));
#3995=DIRECTION('',(0.342020234846066,2.09426992923931E-17,-0.939692587475203));
#3996=DIRECTION('center_axis',(0.148462502781433,0.987440631916705,0.0540359482919519));
#3997=DIRECTION('ref_axis',(-0.927890642383958,0.157990501106673,-0.337724676824699));
#3998=DIRECTION('',(-0.342020234846066,-2.09426992923931E-17,0.939692587475203));
#3999=DIRECTION('',(-0.342020234846066,-2.09426992923931E-17,0.939692587475203));
#4000=DIRECTION('',(-0.927890642383958,0.157990501106673,-0.337724676824699));
#4001=DIRECTION('',(-0.342020234846066,-2.09426992923931E-17,0.939692587475203));
#4002=DIRECTION('center_axis',(0.148462502781433,0.987440631916705,0.0540359482919519));
#4003=DIRECTION('ref_axis',(0.927890642383958,-0.157990501106673,0.337724676824699));
#4004=DIRECTION('',(-0.927890642383958,0.157990501106673,-0.337724676824699));
#4005=DIRECTION('',(-0.342020234846066,-2.09426992923931E-17,0.939692587475203));
#4006=DIRECTION('center_axis',(0.148462502781433,-0.987440631916705,0.0540359482919519));
#4007=DIRECTION('ref_axis',(0.927890642383958,0.157990501106673,0.337724676824699));
#4008=DIRECTION('',(-0.342020234846066,-2.09426992923931E-17,0.939692587475203));
#4009=DIRECTION('',(0.927890642383958,0.157990501106673,0.337724676824699));
#4010=DIRECTION('center_axis',(0.148462502781433,-0.987440631916705,0.0540359482919519));
#4011=DIRECTION('ref_axis',(0.927890642383958,0.157990501106673,0.337724676824699));
#4012=DIRECTION('',(-0.342020234846066,-2.09426992923931E-17,0.939692587475203));
#4013=DIRECTION('',(0.927890642383958,0.157990501106673,0.337724676824699));
#4014=DIRECTION('',(-0.342020234846066,-2.09426992923931E-17,0.939692587475203));
#4015=DIRECTION('',(-0.342020234846066,-2.09426992923931E-17,0.939692587475203));
#4016=DIRECTION('center_axis',(-0.939692587475203,-5.75395759716863E-17,
-0.342020234846066));
#4017=DIRECTION('ref_axis',(6.12323399573548E-17,-1.,-4.78224871431377E-30));
#4018=DIRECTION('',(0.342020234846066,2.09426992923931E-17,-0.939692587475203));
#4019=DIRECTION('',(6.12323399573548E-17,-1.,-4.78224871431377E-30));
#4020=DIRECTION('',(-0.342020234846066,-2.09426992923931E-17,0.939692587475203));
#4021=DIRECTION('',(6.12323399573548E-17,-1.,-4.78224871431377E-30));
#4022=DIRECTION('center_axis',(0.939692587475203,5.75395759716863E-17,0.342020234846066));
#4023=DIRECTION('ref_axis',(-6.12323399573548E-17,1.,4.78224871431377E-30));
#4024=DIRECTION('',(-0.342020234846066,-2.09426992923931E-17,0.939692587475203));
#4025=DIRECTION('',(-6.12323399573548E-17,1.,4.78224871431377E-30));
#4026=DIRECTION('',(0.342020234846066,2.09426992923931E-17,-0.939692587475203));
#4027=DIRECTION('',(-6.12323399573548E-17,1.,4.78224871431377E-30));
#4028=DIRECTION('center_axis',(-0.342020234846066,-2.09426992923931E-17,
0.939692587475203));
#4029=DIRECTION('ref_axis',(0.939692587475203,5.75395759716863E-17,0.342020234846066));
#4030=DIRECTION('',(-0.927890642383958,-0.157990501106673,-0.337724676824699));
#4031=DIRECTION('',(0.927890642383958,-0.157990501106673,0.337724676824699));
#4032=DIRECTION('center_axis',(-6.12323399573548E-17,1.,4.78224871431377E-30));
#4033=DIRECTION('ref_axis',(0.939692587475203,5.75395759716863E-17,0.342020234846066));
#4034=DIRECTION('center_axis',(-6.12323399573548E-17,1.,4.78224871431377E-30));
#4035=DIRECTION('ref_axis',(0.939692587475203,5.75395759716863E-17,0.342020234846066));
#4036=DIRECTION('center_axis',(-6.12323399573548E-17,1.,4.78224871431377E-30));
#4037=DIRECTION('ref_axis',(0.939692587475203,5.75395759716863E-17,0.342020234846066));
#4038=DIRECTION('center_axis',(-6.12323399573548E-17,1.,4.78224871431377E-30));
#4039=DIRECTION('ref_axis',(0.939692587475203,5.75395759716863E-17,0.342020234846066));
#4040=DIRECTION('',(6.12323399573548E-17,-1.,-4.78224871431377E-30));
#4041=DIRECTION('center_axis',(-6.12323399573548E-17,1.,4.78224871431377E-30));
#4042=DIRECTION('ref_axis',(0.939692587475203,5.75395759716863E-17,0.342020234846066));
#4043=DIRECTION('',(-6.12323399573548E-17,1.,4.78224871431377E-30));
#4044=DIRECTION('center_axis',(-6.12323399573548E-17,1.,4.78224871431377E-30));
#4045=DIRECTION('ref_axis',(0.939692587475203,5.75395759716863E-17,0.342020234846066));
#4046=DIRECTION('center_axis',(-6.12323399573548E-17,1.,4.78224871431377E-30));
#4047=DIRECTION('ref_axis',(-0.939692587475203,-5.75395759716863E-17,-0.342020234846066));
#4048=DIRECTION('center_axis',(0.148462502781433,0.987440631916705,0.0540359482919519));
#4049=DIRECTION('ref_axis',(0.927890642383958,-0.157990501106673,0.337724676824699));
#4050=DIRECTION('center_axis',(-0.148462502781433,-0.987440631916705,-0.0540359482919519));
#4051=DIRECTION('ref_axis',(0.927890642383958,-0.157990501106673,0.337724676824699));
#4052=DIRECTION('',(-0.342020234846066,-2.09426992923931E-17,0.939692587475203));
#4053=DIRECTION('',(0.927890642383958,-0.157990501106673,0.337724676824699));
#4054=DIRECTION('',(0.927890642383958,-0.157990501106673,0.337724676824699));
#4055=DIRECTION('',(-0.342020234846066,-2.09426992923931E-17,0.939692587475203));
#4056=DIRECTION('',(0.927890642383958,-0.157990501106673,0.337724676824699));
#4057=DIRECTION('center_axis',(0.939692587475203,5.75395759716863E-17,0.342020234846066));
#4058=DIRECTION('ref_axis',(-6.12323399573548E-17,1.,4.78224871431377E-30));
#4059=DIRECTION('',(-6.12323399573548E-17,1.,4.78224871431377E-30));
#4060=DIRECTION('center_axis',(-0.939692587475203,-5.75395759716863E-17,
-0.342020234846066));
#4061=DIRECTION('ref_axis',(6.12323399573548E-17,-1.,-4.78224871431377E-30));
#4062=DIRECTION('',(6.12323399573548E-17,-1.,-4.78224871431377E-30));
#4063=DIRECTION('',(6.12323399573548E-17,-1.,-4.78224871431377E-30));
#4064=DIRECTION('center_axis',(-0.342020234846066,-2.09426992923931E-17,
0.939692587475203));
#4065=DIRECTION('ref_axis',(0.939692587475203,5.75395759716863E-17,0.342020234846066));
#4066=DIRECTION('',(-6.12323399573548E-17,1.,4.78224871431377E-30));
#4067=DIRECTION('center_axis',(-6.12323399573548E-17,1.,4.78224871431377E-30));
#4068=DIRECTION('ref_axis',(0.939692587475203,5.75395759716863E-17,0.342020234846066));
#4069=DIRECTION('center_axis',(-6.12323399573548E-17,1.,4.78224871431377E-30));
#4070=DIRECTION('ref_axis',(0.939692587475203,5.75395759716863E-17,0.342020234846066));
#4071=DIRECTION('center_axis',(-6.12323399573548E-17,1.,4.78224871431377E-30));
#4072=DIRECTION('ref_axis',(-0.939692587475203,-5.75395759716863E-17,-0.342020234846066));
#4073=DIRECTION('center_axis',(-6.12323399573548E-17,1.,4.78224871431377E-30));
#4074=DIRECTION('ref_axis',(0.939692587475203,5.75395759716863E-17,0.342020234846066));
#4075=DIRECTION('center_axis',(-6.12323399573548E-17,1.,4.78224871431377E-30));
#4076=DIRECTION('ref_axis',(0.939692587475203,5.75395759716863E-17,0.342020234846066));
#4077=DIRECTION('center_axis',(-0.148462502781433,0.987440631916705,-0.0540359482919519));
#4078=DIRECTION('ref_axis',(-0.927890642383958,-0.157990501106673,-0.337724676824699));
#4079=DIRECTION('',(-0.927890642383958,-0.157990501106673,-0.337724676824699));
#4080=DIRECTION('center_axis',(0.148462502781433,-0.987440631916705,0.0540359482919519));
#4081=DIRECTION('ref_axis',(0.927890642383958,0.157990501106673,0.337724676824699));
#4082=DIRECTION('',(-0.342020234846066,-2.09426992923931E-17,0.939692587475203));
#4083=DIRECTION('',(-0.927890642383958,-0.157990501106673,-0.337724676824699));
#4084=DIRECTION('',(-0.927890642383958,-0.157990501106673,-0.337724676824699));
#4085=DIRECTION('',(-0.342020234846066,-2.09426992923931E-17,0.939692587475203));
#4086=DIRECTION('center_axis',(-6.12323399573548E-17,1.,4.78224871431377E-30));
#4087=DIRECTION('ref_axis',(0.939692587475203,5.75395759716863E-17,0.342020234846066));
#4088=DIRECTION('center_axis',(-6.12323399573548E-17,1.,4.78224871431377E-30));
#4089=DIRECTION('ref_axis',(0.939692587475203,5.75395759716863E-17,0.342020234846066));
#4090=DIRECTION('center_axis',(-6.12323399573548E-17,1.,4.78224871431377E-30));
#4091=DIRECTION('ref_axis',(0.939692587475203,5.75395759716863E-17,0.342020234846066));
#4092=DIRECTION('center_axis',(-6.12323399573548E-17,1.,4.78224871431377E-30));
#4093=DIRECTION('ref_axis',(-0.939692587475202,-5.75395759716863E-17,-0.342020234846067));
#4094=DIRECTION('center_axis',(-6.12323399573548E-17,1.,4.78224871431377E-30));
#4095=DIRECTION('ref_axis',(0.939692587475203,5.75395759716863E-17,0.342020234846066));
#4096=DIRECTION('',(6.12323399573548E-17,-1.,-4.78224871431377E-30));
#4097=DIRECTION('',(-6.12323399573548E-17,1.,4.78224871431377E-30));
#4098=DIRECTION('center_axis',(-6.12323399573548E-17,1.,4.78224871431377E-30));
#4099=DIRECTION('ref_axis',(0.939692587475203,5.75395759716863E-17,0.342020234846066));
#4100=DIRECTION('center_axis',(-6.12323399573548E-17,1.,4.78224871431377E-30));
#4101=DIRECTION('ref_axis',(0.939692587475203,5.75395759716863E-17,0.342020234846066));
#4102=DIRECTION('center_axis',(0.939692587475203,5.75395759716863E-17,0.342020234846066));
#4103=DIRECTION('ref_axis',(-6.12323399573548E-17,1.,4.78224871431377E-30));
#4104=DIRECTION('',(-6.12323399573548E-17,1.,4.78224871431377E-30));
#4105=DIRECTION('center_axis',(-0.939692587475203,-5.75395759716863E-17,
-0.342020234846066));
#4106=DIRECTION('ref_axis',(6.12323399573548E-17,-1.,-4.78224871431377E-30));
#4107=DIRECTION('',(6.12323399573548E-17,-1.,-4.78224871431377E-30));
#4108=DIRECTION('',(6.12323399573548E-17,-1.,-4.78224871431377E-30));
#4109=DIRECTION('center_axis',(-0.342020234846066,-2.09426992923931E-17,
0.939692587475203));
#4110=DIRECTION('ref_axis',(0.939692587475203,5.75395759716863E-17,0.342020234846066));
#4111=DIRECTION('',(-6.12323399573548E-17,1.,4.78224871431377E-30));
#4112=DIRECTION('center_axis',(-0.342020234846066,-2.09426992923931E-17,
0.939692587475203));
#4113=DIRECTION('ref_axis',(0.939692587475203,5.75395759716863E-17,0.342020234846066));
#4114=DIRECTION('center_axis',(-6.12323399573548E-17,1.,4.78224871431377E-30));
#4115=DIRECTION('ref_axis',(0.939692587475203,5.75395759716863E-17,0.342020234846066));
#4116=DIRECTION('center_axis',(-6.12323399573548E-17,1.,4.78224871431377E-30));
#4117=DIRECTION('ref_axis',(0.939692587475203,5.75395759716863E-17,0.342020234846066));
#4118=DIRECTION('center_axis',(-6.12323399573548E-17,1.,4.78224871431377E-30));
#4119=DIRECTION('ref_axis',(0.939692587475203,5.75395759716863E-17,0.342020234846066));
#4120=DIRECTION('center_axis',(-6.12323399573548E-17,1.,4.78224871431377E-30));
#4121=DIRECTION('ref_axis',(0.939692587475203,5.75395759716863E-17,0.342020234846066));
#4122=DIRECTION('center_axis',(-6.12323399573548E-17,1.,4.78224871431377E-30));
#4123=DIRECTION('ref_axis',(-0.939692587475203,-5.75395759716863E-17,-0.342020234846066));
#4984=CARTESIAN_POINT('',(0.,0.,0.));
#4985=CARTESIAN_POINT('Origin',(-8.88178419700125E-16,-1.70000000000019,
3.));
#4986=CARTESIAN_POINT('',(-0.385273960864878,-1.52000000000017,2.8597717037131));
#4987=CARTESIAN_POINT('Origin',(-8.88178419700125E-16,-1.52000000000017,
3.));
#4988=CARTESIAN_POINT('',(-0.385273960864878,-1.28000000000015,2.8597717037131));
#4989=CARTESIAN_POINT('',(-0.385273960864878,-1.70000000000019,2.8597717037131));
#4990=CARTESIAN_POINT('',(-0.140228296286904,-1.28000000000015,3.38527396086488));
#4991=CARTESIAN_POINT('Origin',(-8.88178419700125E-16,-1.28000000000015,
3.));
#4992=CARTESIAN_POINT('',(0.140228296286902,-1.28000000000015,2.61472603913512));
#4993=CARTESIAN_POINT('Origin',(-8.88178419700125E-16,-1.28000000000015,
3.));
#4994=CARTESIAN_POINT('Origin',(-8.88178419700125E-16,-1.28000000000015,
3.));
#4995=CARTESIAN_POINT('Origin',(-8.88178419700125E-16,-1.70000000000019,
3.));
#4996=CARTESIAN_POINT('',(-0.140228296286904,1.28000000000015,3.38527396086488));
#4997=CARTESIAN_POINT('',(0.140228296286902,1.28000000000015,2.61472603913512));
#4998=CARTESIAN_POINT('Origin',(-8.88178419700125E-16,1.28000000000015,
3.));
#4999=CARTESIAN_POINT('',(-0.385273960864878,1.28000000000015,2.8597717037131));
#5000=CARTESIAN_POINT('Origin',(-8.88178419700125E-16,1.28000000000015,
3.));
#5001=CARTESIAN_POINT('',(-0.385273960864878,1.52000000000017,2.8597717037131));
#5002=CARTESIAN_POINT('',(-0.385273960864878,-1.70000000000019,2.8597717037131));
#5003=CARTESIAN_POINT('Origin',(-8.88178419700125E-16,1.52000000000017,
3.));
#5004=CARTESIAN_POINT('Origin',(-8.88178419700125E-16,1.28000000000015,
3.));
#5005=CARTESIAN_POINT('Origin',(2.34923146868827,-1.70000000000019,3.85505058711526));
#5006=CARTESIAN_POINT('',(2.20900317240137,-1.12000000000013,4.24032454798014));
#5007=CARTESIAN_POINT('',(2.48945976497518,-1.12000000000013,3.46977662625038));
#5008=CARTESIAN_POINT('Origin',(2.34923146868827,-1.12000000000013,3.85505058711526));
#5009=CARTESIAN_POINT('',(1.9639575078234,-1.18560000000013,3.71482229082836));
#5010=CARTESIAN_POINT('Origin',(2.34923146868827,-1.12000000000013,3.85505058711526));
#5011=CARTESIAN_POINT('',(1.9639575078234,-0.8800000000001,3.71482229082836));
#5012=CARTESIAN_POINT('',(1.9639575078234,-1.70000000000019,3.71482229082836));
#5013=CARTESIAN_POINT('Origin',(2.34923146868827,-0.8800000000001,3.85505058711526));
#5014=CARTESIAN_POINT('Origin',(2.34923146868827,-1.12000000000013,3.85505058711526));
#5015=CARTESIAN_POINT('Origin',(2.34923146868827,-1.70000000000019,3.85505058711526));
#5016=CARTESIAN_POINT('',(1.9639575078234,0.8800000000001,3.71482229082836));
#5017=CARTESIAN_POINT('Origin',(2.34923146868827,0.8800000000001,3.85505058711526));
#5018=CARTESIAN_POINT('',(1.9639575078234,1.18560000000014,3.71482229082836));
#5019=CARTESIAN_POINT('',(1.9639575078234,-1.70000000000019,3.71482229082836));
#5020=CARTESIAN_POINT('',(2.20900317240137,1.12000000000013,4.24032454798014));
#5021=CARTESIAN_POINT('Origin',(2.34923146868827,1.12000000000013,3.85505058711526));
#5022=CARTESIAN_POINT('',(2.48945976497518,1.12000000000013,3.46977662625038));
#5023=CARTESIAN_POINT('Origin',(2.34923146868827,1.12000000000013,3.85505058711526));
#5024=CARTESIAN_POINT('Origin',(2.34923146868827,1.12000000000013,3.85505058711526));
#5025=CARTESIAN_POINT('Origin',(-8.88178419700125E-16,1.28000000000015,
3.));
#5026=CARTESIAN_POINT('',(-0.239414164392274,1.28000000000015,3.65778481123272));
#5027=CARTESIAN_POINT('',(0.342020234846104,1.28000000000015,2.06030741252469));
#5028=CARTESIAN_POINT('',(0.239414164392272,1.28000000000015,2.34221518876728));
#5029=CARTESIAN_POINT('Origin',(-8.88178419700125E-16,1.28000000000015,
3.));
#5030=CARTESIAN_POINT('',(0.342020234846104,1.28000000000015,2.06030741252469));
#5031=CARTESIAN_POINT('Origin',(-8.88178419700125E-16,-1.28000000000015,
3.));
#5032=CARTESIAN_POINT('',(0.239414164392273,-1.28000000000015,2.34221518876728));
#5033=CARTESIAN_POINT('',(0.342020234846104,-1.28000000000015,2.06030741252469));
#5034=CARTESIAN_POINT('',(-0.239414164392274,-1.28000000000015,3.65778481123272));
#5035=CARTESIAN_POINT('Origin',(-8.88178419700125E-16,-1.28000000000015,
3.));
#5036=CARTESIAN_POINT('',(0.342020234846104,-1.28000000000015,2.06030741252469));
#5037=CARTESIAN_POINT('Origin',(3.03327193838048,1.12000000000013,1.97566541216464));
#5038=CARTESIAN_POINT('',(2.58864563308055,1.12000000000013,3.19726577588254));
#5039=CARTESIAN_POINT('',(3.03327193838048,1.12000000000013,1.97566541216464));
#5040=CARTESIAN_POINT('',(3.03327193838048,1.12000000000013,1.97566541216464));
#5041=CARTESIAN_POINT('',(3.03327193838048,1.12000000000013,1.97566541216464));
#5042=CARTESIAN_POINT('',(0.684040469692209,1.52000000000017,1.12061482504938));
#5043=CARTESIAN_POINT('',(3.03327193838048,1.12000000000013,1.97566541216464));
#5044=CARTESIAN_POINT('',(0.239414164392272,1.52000000000017,2.34221518876728));
#5045=CARTESIAN_POINT('',(0.684040469692209,1.52000000000017,1.12061482504938));
#5046=CARTESIAN_POINT('',(-0.239414164392274,1.52000000000017,3.65778481123272));
#5047=CARTESIAN_POINT('Origin',(-8.88178419700125E-16,1.52000000000017,
3.));
#5048=CARTESIAN_POINT('',(2.109817304296,1.12000000000013,4.51283539834798));
#5049=CARTESIAN_POINT('',(2.109817304296,1.12000000000013,4.51283539834798));
#5050=CARTESIAN_POINT('',(3.03327193838048,1.12000000000013,1.97566541216464));
#5051=CARTESIAN_POINT('Origin',(0.684040469692209,-1.52000000000017,1.12061482504938));
#5052=CARTESIAN_POINT('',(2.109817304296,-1.12000000000013,4.51283539834798));
#5053=CARTESIAN_POINT('',(3.03327193838048,-1.12000000000013,1.97566541216464));
#5054=CARTESIAN_POINT('',(-0.239414164392274,-1.52000000000017,3.65778481123272));
#5055=CARTESIAN_POINT('',(-0.239414164392274,-1.52000000000017,3.65778481123272));
#5056=CARTESIAN_POINT('',(0.239414164392273,-1.52000000000017,2.34221518876728));
#5057=CARTESIAN_POINT('Origin',(-8.88178419700125E-16,-1.52000000000017,
3.));
#5058=CARTESIAN_POINT('',(0.684040469692209,-1.52000000000017,1.12061482504938));
#5059=CARTESIAN_POINT('',(0.684040469692209,-1.52000000000017,1.12061482504938));
#5060=CARTESIAN_POINT('',(3.03327193838048,-1.12000000000013,1.97566541216464));
#5061=CARTESIAN_POINT('',(0.684040469692209,-1.52000000000017,1.12061482504938));
#5062=CARTESIAN_POINT('',(2.58864563308055,-1.12000000000013,3.19726577588255));
#5063=CARTESIAN_POINT('',(3.03327193838048,-1.12000000000013,1.97566541216464));
#5064=CARTESIAN_POINT('',(3.03327193838048,-1.12000000000013,1.97566541216464));
#5065=CARTESIAN_POINT('Origin',(1.43579453967246,1.30000000000015,1.39423101292626));
#5066=CARTESIAN_POINT('',(1.33318846921863,-1.15200000000013,1.67613878916886));
#5067=CARTESIAN_POINT('',(1.43579453967246,-1.15200000000013,1.39423101292626));
#5068=CARTESIAN_POINT('',(1.43579453967246,-1.15200000000013,1.39423101292626));
#5069=CARTESIAN_POINT('',(1.33318846921863,1.15200000000013,1.67613878916886));
#5070=CARTESIAN_POINT('',(1.33318846921863,1.30000000000015,1.67613878916886));
#5071=CARTESIAN_POINT('',(1.43579453967246,1.15200000000013,1.39423101292626));
#5072=CARTESIAN_POINT('',(1.43579453967246,1.15200000000013,1.39423101292626));
#5073=CARTESIAN_POINT('',(1.43579453967246,1.30000000000015,1.39423101292626));
#5074=CARTESIAN_POINT('Origin',(2.28151786840024,-1.15000000000013,1.70204922428776));
#5075=CARTESIAN_POINT('',(2.28151786840024,-1.00800000000012,1.70204922428776));
#5076=CARTESIAN_POINT('',(2.17891179794641,-1.00800000000012,1.98395700053035));
#5077=CARTESIAN_POINT('',(2.28151786840024,-1.00800000000012,1.70204922428776));
#5078=CARTESIAN_POINT('',(2.28151786840024,1.00800000000012,1.70204922428776));
#5079=CARTESIAN_POINT('',(2.28151786840024,-1.15000000000013,1.70204922428776));
#5080=CARTESIAN_POINT('',(2.17891179794641,1.00800000000012,1.98395700053035));
#5081=CARTESIAN_POINT('',(2.28151786840024,1.00800000000012,1.70204922428776));
#5082=CARTESIAN_POINT('',(2.17891179794641,-1.15000000000013,1.98395700053035));
#5083=CARTESIAN_POINT('Origin',(1.75605013358252,1.07527058761815E-16,1.8300478948496));
#5084=CARTESIAN_POINT('',(2.42252087083831,-0.966521060842544,2.07262347872934));
#5085=CARTESIAN_POINT('',(1.24790513649417,1.16652106084257,1.64509818517171));
#5086=CARTESIAN_POINT('Origin',(2.34923146868827,0.880000000000101,3.85505058711526));
#5087=CARTESIAN_POINT('',(2.58864563308055,0.880000000000101,3.19726577588255));
#5088=CARTESIAN_POINT('',(2.109817304296,0.880000000000101,4.51283539834798));
#5089=CARTESIAN_POINT('Origin',(2.34923146868827,0.880000000000101,3.85505058711526));
#5090=CARTESIAN_POINT('Origin',(2.34923146868827,0.880000000000101,3.85505058711526));
#5091=CARTESIAN_POINT('Origin',(2.34923146868827,0.880000000000101,3.85505058711526));
#5092=CARTESIAN_POINT('',(2.58864563308055,0.880000000000101,3.19726577588255));
#5093=CARTESIAN_POINT('Origin',(2.34923146868827,1.12000000000013,3.85505058711526));
#5094=CARTESIAN_POINT('',(2.109817304296,0.880000000000101,4.51283539834798));
#5095=CARTESIAN_POINT('Origin',(2.34923146868827,1.12000000000013,3.85505058711526));
#5096=CARTESIAN_POINT('Origin',(2.34923146868827,0.880000000000101,3.85505058711526));
#5097=CARTESIAN_POINT('Origin',(2.34923146868827,0.880000000000101,3.85505058711526));
#5098=CARTESIAN_POINT('Origin',(0.684040469692209,1.28000000000015,1.12061482504938));
#5099=CARTESIAN_POINT('',(0.684040469692209,1.28000000000015,1.12061482504938));
#5100=CARTESIAN_POINT('',(0.684040469692209,1.28000000000015,1.12061482504938));
#5101=CARTESIAN_POINT('',(0.684040469692209,1.28000000000015,1.12061482504938));
#5102=CARTESIAN_POINT('',(3.03327193838048,0.880000000000101,1.97566541216464));
#5103=CARTESIAN_POINT('',(0.684040469692209,1.28000000000015,1.12061482504938));
#5104=CARTESIAN_POINT('',(3.03327193838048,0.880000000000101,1.97566541216464));
#5105=CARTESIAN_POINT('',(-0.239414164392274,1.28000000000015,3.65778481123272));
#5106=CARTESIAN_POINT('Origin',(3.03327193838048,0.880000000000101,1.97566541216464));
#5107=CARTESIAN_POINT('',(3.03327193838048,0.880000000000101,1.97566541216464));
#5108=CARTESIAN_POINT('Origin',(0.684040469692209,1.52000000000017,1.12061482504938));
#5109=CARTESIAN_POINT('',(0.239414164392272,1.28000000000015,2.34221518876728));
#5110=CARTESIAN_POINT('',(0.684040469692209,1.52000000000017,1.12061482504938));
#5111=CARTESIAN_POINT('Origin',(0.935201569951863,1.20000000000014,4.08531010479035));
#5112=CARTESIAN_POINT('',(-0.239414164392274,1.28000000000015,3.65778481123272));
#5113=CARTESIAN_POINT('Origin',(-8.88178419700125E-16,1.28000000000015,
3.));
#5114=CARTESIAN_POINT('Origin',(-8.88178419700125E-16,1.52000000000017,
3.));
#5115=CARTESIAN_POINT('Origin',(-8.88178419700125E-16,1.28000000000015,
3.));
#5116=CARTESIAN_POINT('Origin',(-8.88178419700125E-16,1.52000000000017,
3.));
#5117=CARTESIAN_POINT('Origin',(-8.88178419700125E-16,1.52000000000017,
3.));
#5118=CARTESIAN_POINT('Origin',(3.03327193838048,-0.8800000000001,1.97566541216464));
#5119=CARTESIAN_POINT('',(2.109817304296,-0.8800000000001,4.51283539834798));
#5120=CARTESIAN_POINT('',(2.109817304296,-0.8800000000001,4.51283539834798));
#5121=CARTESIAN_POINT('',(2.58864563308055,-0.8800000000001,3.19726577588255));
#5122=CARTESIAN_POINT('Origin',(2.34923146868827,-0.8800000000001,3.85505058711526));
#5123=CARTESIAN_POINT('',(3.03327193838048,-0.8800000000001,1.97566541216464));
#5124=CARTESIAN_POINT('',(3.03327193838048,-0.8800000000001,1.97566541216464));
#5125=CARTESIAN_POINT('',(3.03327193838048,-0.8800000000001,1.97566541216464));
#5126=CARTESIAN_POINT('',(0.684040469692209,-1.28000000000015,1.12061482504938));
#5127=CARTESIAN_POINT('',(3.03327193838048,-0.8800000000001,1.97566541216464));
#5128=CARTESIAN_POINT('',(0.684040469692209,-1.28000000000015,1.12061482504938));
#5129=CARTESIAN_POINT('Origin',(2.34923146868827,-0.8800000000001,3.85505058711526));
#5130=CARTESIAN_POINT('Origin',(2.34923146868827,-0.8800000000001,3.85505058711526));
#5131=CARTESIAN_POINT('Origin',(2.34923146868827,-0.8800000000001,3.85505058711526));
#5132=CARTESIAN_POINT('Origin',(2.34923146868827,-1.12000000000013,3.85505058711526));
#5133=CARTESIAN_POINT('Origin',(2.34923146868827,-1.12000000000013,3.85505058711526));
#5134=CARTESIAN_POINT('',(2.58864563308055,-1.12000000000013,3.19726577588255));
#5135=CARTESIAN_POINT('',(2.109817304296,-1.12000000000013,4.51283539834798));
#5136=CARTESIAN_POINT('Origin',(2.34923146868827,-1.12000000000013,3.85505058711526));
#5137=CARTESIAN_POINT('Origin',(2.34923146868827,-1.12000000000013,3.85505058711526));
#5138=CARTESIAN_POINT('Origin',(3.03327193838048,-1.12000000000013,1.97566541216464));
#5139=CARTESIAN_POINT('',(3.03327193838048,-1.12000000000013,1.97566541216464));
#5140=CARTESIAN_POINT('Origin',(0.684040469692209,-1.28000000000015,1.12061482504938));
#5141=CARTESIAN_POINT('',(0.239414164392273,-1.52000000000017,2.34221518876728));
#5142=CARTESIAN_POINT('',(0.684040469692209,-1.28000000000015,1.12061482504938));
#5143=CARTESIAN_POINT('Origin',(0.935201569951863,-1.20000000000014,4.08531010479035));
#5144=CARTESIAN_POINT('',(-0.239414164392274,-1.52000000000017,3.65778481123272));
#5145=CARTESIAN_POINT('Origin',(1.85865620403635,-1.20000000000014,1.54814011860701));
#5146=CARTESIAN_POINT('Origin',(-8.88178419700125E-16,-1.52000000000017,
3.));
#5147=CARTESIAN_POINT('Origin',(-8.88178419700125E-16,-1.52000000000017,
3.));
#5148=CARTESIAN_POINT('Origin',(-8.88178419700125E-16,-1.52000000000017,
3.));
#5149=CARTESIAN_POINT('Origin',(-8.88178419700125E-16,-1.52000000000017,
3.));
#5150=CARTESIAN_POINT('Origin',(-8.88178419700125E-16,-1.52000000000017,
3.));
#5886=UNCERTAINTY_MEASURE_WITH_UNIT(LENGTH_MEASURE(0.001),#5930,
'DISTANCE_ACCURACY_VALUE',
'Maximum model space distance between geometric entities at asserted c
onnectivities');
#5905=UNCERTAINTY_MEASURE_WITH_UNIT(LENGTH_MEASURE(0.001),#5930,
'DISTANCE_ACCURACY_VALUE',
'Maximum model space distance between geometric entities at asserted c
onnectivities');
#5910=(
GEOMETRIC_REPRESENTATION_CONTEXT(3)
GLOBAL_UNCERTAINTY_ASSIGNED_CONTEXT((#5886))
GLOBAL_UNIT_ASSIGNED_CONTEXT((#5930,#5932,#5933))
REPRESENTATION_CONTEXT('','3D')
);
#5929=(
GEOMETRIC_REPRESENTATION_CONTEXT(3)
GLOBAL_UNCERTAINTY_ASSIGNED_CONTEXT((#5905))
GLOBAL_UNIT_ASSIGNED_CONTEXT((#5930,#5932,#5933))
REPRESENTATION_CONTEXT('','3D')
);
#5930=(
LENGTH_UNIT()
NAMED_UNIT(*)
SI_UNIT(.CENTI.,.METRE.)
);
#5932=(
NAMED_UNIT(*)
PLANE_ANGLE_UNIT()
SI_UNIT($,.RADIAN.)
);
#5933=(
NAMED_UNIT(*)
SI_UNIT($,.STERADIAN.)
SOLID_ANGLE_UNIT()
);
#5938=SHAPE_DEFINITION_REPRESENTATION(#5961,#6043);
#5961=PRODUCT_DEFINITION_SHAPE('',$,#6067);
#6043=SHAPE_REPRESENTATION('',(#3460),#5910);
#6062=PRODUCT_DEFINITION_CONTEXT('part definition',#6133,'design');
#6067=PRODUCT_DEFINITION('Offset cable chain link',
'Offset cable chain link',#6090,#6062);
#6090=PRODUCT_DEFINITION_FORMATION('',$,#6139);
#6133=APPLICATION_CONTEXT(
'Core Data for Automotive Mechanical Design Process');
#6134=PRODUCT_CONTEXT('part definition',#6133,'mechanical');
#6139=PRODUCT('Offset cable chain link','Offset cable chain link',
'Offset cable chain link',(#6134));
#6228=COLOUR_RGB('Off White',0.89,0.88,0.83);
#6229=FILL_AREA_STYLE_COLOUR('',#6228);
#6230=FILL_AREA_STYLE('',(#6229));
#6231=SURFACE_STYLE_FILL_AREA(#6230);
#6232=SURFACE_SIDE_STYLE('',(#6231));
#6233=SURFACE_STYLE_USAGE(.BOTH.,#6232);
#6234=PRESENTATION_STYLE_ASSIGNMENT((#6233));
ENDSEC;
END-ISO-10303-21;
